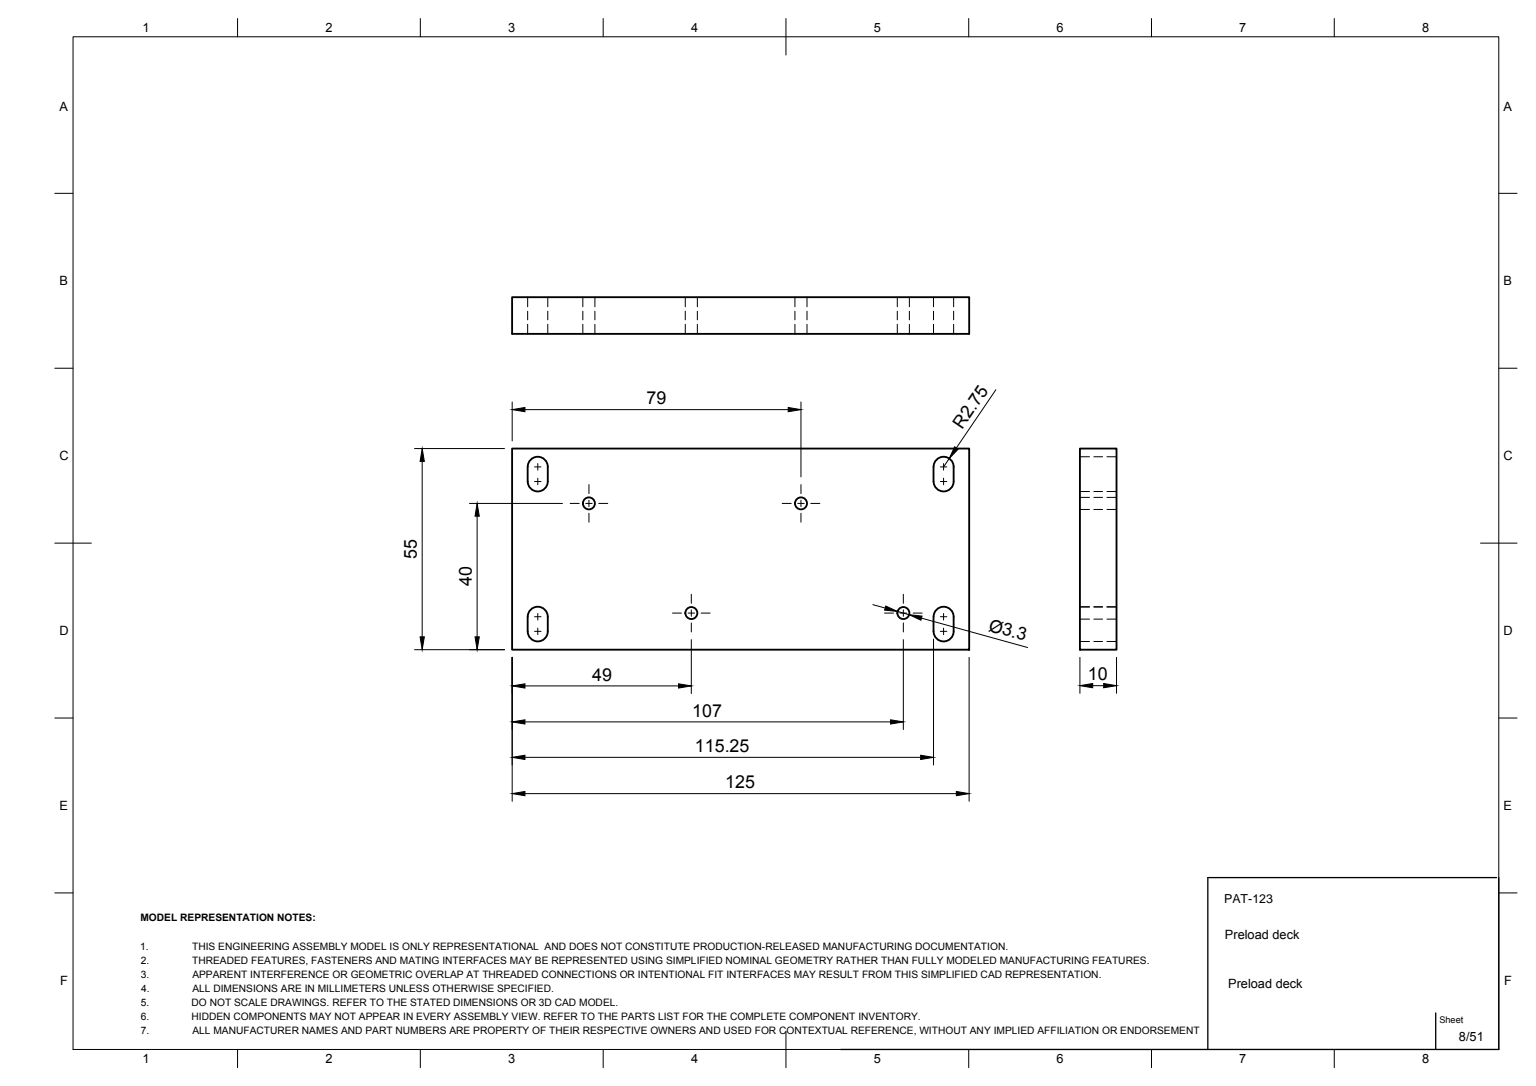
ISO-10303-21;
HEADER;
/* Generated by software containing ST-Developer
 * from STEP Tools, Inc. (www.steptools.com) 
 */

FILE_DESCRIPTION(
/* description */ ('Worm-less right-angle friction wheel drive'),
/* implementation_level */ '2;1');

FILE_NAME(
/* name */ 'Preload deck.step',
/* time_stamp */ '2026-10-28T03:22:36-07:00',
/* author */ (''),
/* organization */ (''),
/* preprocessor_version */ 'ST-DEVELOPER v20.2',
/* originating_system */ 'Autodesk Translation Framework v15.17.0.0',
/* authorisation */ '');

FILE_SCHEMA (('AUTOMOTIVE_DESIGN { 1 0 10303 214 3 1 1 }'));
ENDSEC;

DATA;
#10=MECHANICAL_DESIGN_GEOMETRIC_PRESENTATION_REPRESENTATION('',(#614),#17046);
#520=SHAPE_REPRESENTATION_RELATIONSHIP('SRR','None',#17263,#567);
#567=ADVANCED_BREP_SHAPE_REPRESENTATION('',(#668),#16999);
#614=STYLED_ITEM('',(#17584),#668);
#668=MANIFOLD_SOLID_BREP('Body1',#8169);
#735=FACE_BOUND('',#1729,.T.);
#736=FACE_BOUND('',#1730,.T.);
#737=FACE_BOUND('',#1731,.T.);
#738=FACE_BOUND('',#1732,.T.);
#739=FACE_BOUND('',#1733,.T.);
#740=FACE_BOUND('',#1734,.T.);
#741=FACE_BOUND('',#1735,.T.);
#742=FACE_BOUND('',#1736,.T.);
#743=FACE_BOUND('',#1756,.T.);
#744=FACE_BOUND('',#1757,.T.);
#745=FACE_BOUND('',#1758,.T.);
#746=FACE_BOUND('',#1759,.T.);
#747=FACE_BOUND('',#1760,.T.);
#748=FACE_BOUND('',#1761,.T.);
#749=FACE_BOUND('',#1762,.T.);
#750=FACE_BOUND('',#1763,.T.);
#970=PLANE('',#8814);
#971=PLANE('',#8821);
#972=PLANE('',#8822);
#973=PLANE('',#8827);
#974=PLANE('',#8828);
#975=PLANE('',#8833);
#976=PLANE('',#8834);
#977=PLANE('',#8839);
#978=PLANE('',#8840);
#979=PLANE('',#8841);
#980=PLANE('',#8842);
#981=PLANE('',#8843);
#982=PLANE('',#8844);
#983=PLANE('',#8845);
#1236=FACE_OUTER_BOUND('',#1722,.T.);
#1237=FACE_OUTER_BOUND('',#1723,.T.);
#1238=FACE_OUTER_BOUND('',#1724,.T.);
#1239=FACE_OUTER_BOUND('',#1725,.T.);
#1240=FACE_OUTER_BOUND('',#1726,.T.);
#1241=FACE_OUTER_BOUND('',#1727,.T.);
#1242=FACE_OUTER_BOUND('',#1728,.T.);
#1243=FACE_OUTER_BOUND('',#1737,.T.);
#1244=FACE_OUTER_BOUND('',#1738,.T.);
#1245=FACE_OUTER_BOUND('',#1739,.T.);
#1246=FACE_OUTER_BOUND('',#1740,.T.);
#1247=FACE_OUTER_BOUND('',#1741,.T.);
#1248=FACE_OUTER_BOUND('',#1742,.T.);
#1249=FACE_OUTER_BOUND('',#1743,.T.);
#1250=FACE_OUTER_BOUND('',#1744,.T.);
#1251=FACE_OUTER_BOUND('',#1745,.T.);
#1252=FACE_OUTER_BOUND('',#1746,.T.);
#1253=FACE_OUTER_BOUND('',#1747,.T.);
#1254=FACE_OUTER_BOUND('',#1748,.T.);
#1255=FACE_OUTER_BOUND('',#1749,.T.);
#1256=FACE_OUTER_BOUND('',#1750,.T.);
#1257=FACE_OUTER_BOUND('',#1751,.T.);
#1258=FACE_OUTER_BOUND('',#1752,.T.);
#1259=FACE_OUTER_BOUND('',#1753,.T.);
#1260=FACE_OUTER_BOUND('',#1754,.T.);
#1261=FACE_OUTER_BOUND('',#1755,.T.);
#1722=EDGE_LOOP('',(#5666,#5667,#5668,#5669));
#1723=EDGE_LOOP('',(#5670,#5671,#5672,#5673));
#1724=EDGE_LOOP('',(#5674,#5675,#5676,#5677));
#1725=EDGE_LOOP('',(#5678,#5679,#5680,#5681));
#1726=EDGE_LOOP('',(#5682,#5683,#5684,#5685));
#1727=EDGE_LOOP('',(#5686,#5687,#5688,#5689));
#1728=EDGE_LOOP('',(#5690,#5691,#5692,#5693));
#1729=EDGE_LOOP('',(#5694,#5695,#5696,#5697));
#1730=EDGE_LOOP('',(#5698,#5699,#5700,#5701));
#1731=EDGE_LOOP('',(#5702,#5703,#5704,#5705));
#1732=EDGE_LOOP('',(#5706,#5707,#5708,#5709));
#1733=EDGE_LOOP('',(#5710));
#1734=EDGE_LOOP('',(#5711));
#1735=EDGE_LOOP('',(#5712));
#1736=EDGE_LOOP('',(#5713));
#1737=EDGE_LOOP('',(#5714,#5715,#5716,#5717));
#1738=EDGE_LOOP('',(#5718,#5719,#5720,#5721));
#1739=EDGE_LOOP('',(#5722,#5723,#5724,#5725));
#1740=EDGE_LOOP('',(#5726,#5727,#5728,#5729));
#1741=EDGE_LOOP('',(#5730,#5731,#5732,#5733));
#1742=EDGE_LOOP('',(#5734,#5735,#5736,#5737));
#1743=EDGE_LOOP('',(#5738,#5739,#5740,#5741));
#1744=EDGE_LOOP('',(#5742,#5743,#5744,#5745));
#1745=EDGE_LOOP('',(#5746,#5747,#5748,#5749));
#1746=EDGE_LOOP('',(#5750,#5751,#5752,#5753));
#1747=EDGE_LOOP('',(#5754,#5755,#5756,#5757));
#1748=EDGE_LOOP('',(#5758,#5759,#5760,#5761));
#1749=EDGE_LOOP('',(#5762,#5763,#5764,#5765));
#1750=EDGE_LOOP('',(#5766,#5767,#5768,#5769));
#1751=EDGE_LOOP('',(#5770,#5771,#5772,#5773));
#1752=EDGE_LOOP('',(#5774,#5775,#5776,#5777));
#1753=EDGE_LOOP('',(#5778,#5779,#5780,#5781));
#1754=EDGE_LOOP('',(#5782,#5783,#5784,#5785));
#1755=EDGE_LOOP('',(#5786,#5787,#5788,#5789));
#1756=EDGE_LOOP('',(#5790,#5791,#5792,#5793));
#1757=EDGE_LOOP('',(#5794,#5795,#5796,#5797));
#1758=EDGE_LOOP('',(#5798,#5799,#5800,#5801));
#1759=EDGE_LOOP('',(#5802,#5803,#5804,#5805));
#1760=EDGE_LOOP('',(#5806));
#1761=EDGE_LOOP('',(#5807));
#1762=EDGE_LOOP('',(#5808));
#1763=EDGE_LOOP('',(#5809));
#2423=LINE('',#12523,#2963);
#2424=LINE('',#12529,#2964);
#2425=LINE('',#12535,#2965);
#2426=LINE('',#12541,#2966);
#2427=LINE('',#12546,#2967);
#2428=LINE('',#12550,#2968);
#2429=LINE('',#12555,#2969);
#2430=LINE('',#12559,#2970);
#2431=LINE('',#12564,#2971);
#2432=LINE('',#12566,#2972);
#2433=LINE('',#12568,#2973);
#2434=LINE('',#12569,#2974);
#2435=LINE('',#12570,#2975);
#2436=LINE('',#12571,#2976);
#2437=LINE('',#12576,#2977);
#2438=LINE('',#12579,#2978);
#2439=LINE('',#12584,#2979);
#2440=LINE('',#12587,#2980);
#2441=LINE('',#12592,#2981);
#2442=LINE('',#12595,#2982);
#2443=LINE('',#12597,#2983);
#2444=LINE('',#12599,#2984);
#2445=LINE('',#12602,#2985);
#2446=LINE('',#12604,#2986);
#2447=LINE('',#12608,#2987);
#2448=LINE('',#12610,#2988);
#2449=LINE('',#12613,#2989);
#2450=LINE('',#12615,#2990);
#2451=LINE('',#12618,#2991);
#2452=LINE('',#12620,#2992);
#2453=LINE('',#12624,#2993);
#2454=LINE('',#12626,#2994);
#2455=LINE('',#12629,#2995);
#2456=LINE('',#12631,#2996);
#2457=LINE('',#12634,#2997);
#2458=LINE('',#12636,#2998);
#2459=LINE('',#12640,#2999);
#2460=LINE('',#12642,#3000);
#2461=LINE('',#12645,#3001);
#2462=LINE('',#12647,#3002);
#2463=LINE('',#12651,#3003);
#2464=LINE('',#12652,#3004);
#2465=LINE('',#12653,#3005);
#2466=LINE('',#12656,#3006);
#2467=LINE('',#12657,#3007);
#2468=LINE('',#12660,#3008);
#2469=LINE('',#12661,#3009);
#2470=LINE('',#12663,#3010);
#2963=VECTOR('',#9931,0.165);
#2964=VECTOR('',#9938,0.165);
#2965=VECTOR('',#9945,0.165);
#2966=VECTOR('',#9952,0.165);
#2967=VECTOR('',#9957,1.);
#2968=VECTOR('',#9960,1.);
#2969=VECTOR('',#9965,1.);
#2970=VECTOR('',#9968,1.);
#2971=VECTOR('',#9973,1.);
#2972=VECTOR('',#9974,1.);
#2973=VECTOR('',#9975,1.);
#2974=VECTOR('',#9976,1.);
#2975=VECTOR('',#9977,1.);
#2976=VECTOR('',#9978,1.);
#2977=VECTOR('',#9981,1.);
#2978=VECTOR('',#9984,1.);
#2979=VECTOR('',#9987,1.);
#2980=VECTOR('',#9990,1.);
#2981=VECTOR('',#9993,1.);
#2982=VECTOR('',#9996,1.);
#2983=VECTOR('',#9999,1.);
#2984=VECTOR('',#10002,1.);
#2985=VECTOR('',#10005,1.);
#2986=VECTOR('',#10006,1.);
#2987=VECTOR('',#10011,1.);
#2988=VECTOR('',#10012,1.);
#2989=VECTOR('',#10017,1.);
#2990=VECTOR('',#10020,1.);
#2991=VECTOR('',#10023,1.);
#2992=VECTOR('',#10024,1.);
#2993=VECTOR('',#10029,1.);
#2994=VECTOR('',#10030,1.);
#2995=VECTOR('',#10035,1.);
#2996=VECTOR('',#10038,1.);
#2997=VECTOR('',#10041,1.);
#2998=VECTOR('',#10042,1.);
#2999=VECTOR('',#10047,1.);
#3000=VECTOR('',#10048,1.);
#3001=VECTOR('',#10053,1.);
#3002=VECTOR('',#10056,1.);
#3003=VECTOR('',#10059,1.);
#3004=VECTOR('',#10060,1.);
#3005=VECTOR('',#10061,1.);
#3006=VECTOR('',#10064,1.);
#3007=VECTOR('',#10065,1.);
#3008=VECTOR('',#10068,1.);
#3009=VECTOR('',#10069,1.);
#3010=VECTOR('',#10072,1.);
#3477=CIRCLE('',#8797,0.165);
#3478=CIRCLE('',#8798,0.165);
#3479=CIRCLE('',#8800,0.165);
#3480=CIRCLE('',#8801,0.165);
#3481=CIRCLE('',#8803,0.165);
#3482=CIRCLE('',#8804,0.165);
#3483=CIRCLE('',#8806,0.165);
#3484=CIRCLE('',#8807,0.165);
#3485=CIRCLE('',#8809,0.275);
#3486=CIRCLE('',#8810,0.275);
#3487=CIRCLE('',#8812,0.275);
#3488=CIRCLE('',#8813,0.275);
#3489=CIRCLE('',#8815,0.275);
#3490=CIRCLE('',#8816,0.275);
#3491=CIRCLE('',#8817,0.275);
#3492=CIRCLE('',#8818,0.275);
#3493=CIRCLE('',#8819,0.275);
#3494=CIRCLE('',#8820,0.275);
#3495=CIRCLE('',#8824,0.275);
#3496=CIRCLE('',#8826,0.275);
#3497=CIRCLE('',#8830,0.275);
#3498=CIRCLE('',#8832,0.275);
#3499=CIRCLE('',#8836,0.275);
#3500=CIRCLE('',#8838,0.275);
#3913=VERTEX_POINT('',#12520);
#3914=VERTEX_POINT('',#12522);
#3915=VERTEX_POINT('',#12526);
#3916=VERTEX_POINT('',#12528);
#3917=VERTEX_POINT('',#12532);
#3918=VERTEX_POINT('',#12534);
#3919=VERTEX_POINT('',#12538);
#3920=VERTEX_POINT('',#12540);
#3921=VERTEX_POINT('',#12544);
#3922=VERTEX_POINT('',#12545);
#3923=VERTEX_POINT('',#12547);
#3924=VERTEX_POINT('',#12549);
#3925=VERTEX_POINT('',#12553);
#3926=VERTEX_POINT('',#12554);
#3927=VERTEX_POINT('',#12556);
#3928=VERTEX_POINT('',#12558);
#3929=VERTEX_POINT('',#12562);
#3930=VERTEX_POINT('',#12563);
#3931=VERTEX_POINT('',#12565);
#3932=VERTEX_POINT('',#12567);
#3933=VERTEX_POINT('',#12572);
#3934=VERTEX_POINT('',#12573);
#3935=VERTEX_POINT('',#12575);
#3936=VERTEX_POINT('',#12577);
#3937=VERTEX_POINT('',#12580);
#3938=VERTEX_POINT('',#12581);
#3939=VERTEX_POINT('',#12583);
#3940=VERTEX_POINT('',#12585);
#3941=VERTEX_POINT('',#12588);
#3942=VERTEX_POINT('',#12589);
#3943=VERTEX_POINT('',#12591);
#3944=VERTEX_POINT('',#12593);
#3945=VERTEX_POINT('',#12601);
#3946=VERTEX_POINT('',#12603);
#3947=VERTEX_POINT('',#12607);
#3948=VERTEX_POINT('',#12609);
#3949=VERTEX_POINT('',#12617);
#3950=VERTEX_POINT('',#12619);
#3951=VERTEX_POINT('',#12623);
#3952=VERTEX_POINT('',#12625);
#3953=VERTEX_POINT('',#12633);
#3954=VERTEX_POINT('',#12635);
#3955=VERTEX_POINT('',#12639);
#3956=VERTEX_POINT('',#12641);
#3957=VERTEX_POINT('',#12649);
#3958=VERTEX_POINT('',#12650);
#3959=VERTEX_POINT('',#12655);
#3960=VERTEX_POINT('',#12659);
#4602=EDGE_CURVE('',#3913,#3913,#3477,.T.);
#4603=EDGE_CURVE('',#3913,#3914,#2423,.T.);
#4604=EDGE_CURVE('',#3914,#3914,#3478,.T.);
#4605=EDGE_CURVE('',#3915,#3915,#3479,.T.);
#4606=EDGE_CURVE('',#3915,#3916,#2424,.T.);
#4607=EDGE_CURVE('',#3916,#3916,#3480,.T.);
#4608=EDGE_CURVE('',#3917,#3917,#3481,.T.);
#4609=EDGE_CURVE('',#3917,#3918,#2425,.T.);
#4610=EDGE_CURVE('',#3918,#3918,#3482,.T.);
#4611=EDGE_CURVE('',#3919,#3919,#3483,.T.);
#4612=EDGE_CURVE('',#3919,#3920,#2426,.T.);
#4613=EDGE_CURVE('',#3920,#3920,#3484,.T.);
#4614=EDGE_CURVE('',#3921,#3922,#2427,.T.);
#4615=EDGE_CURVE('',#3923,#3922,#3485,.T.);
#4616=EDGE_CURVE('',#3924,#3923,#2428,.T.);
#4617=EDGE_CURVE('',#3921,#3924,#3486,.T.);
#4618=EDGE_CURVE('',#3925,#3926,#2429,.T.);
#4619=EDGE_CURVE('',#3927,#3926,#3487,.T.);
#4620=EDGE_CURVE('',#3928,#3927,#2430,.T.);
#4621=EDGE_CURVE('',#3925,#3928,#3488,.T.);
#4622=EDGE_CURVE('',#3929,#3930,#2431,.T.);
#4623=EDGE_CURVE('',#3930,#3931,#2432,.T.);
#4624=EDGE_CURVE('',#3931,#3932,#2433,.T.);
#4625=EDGE_CURVE('',#3932,#3929,#2434,.T.);
#4626=EDGE_CURVE('',#3922,#3927,#2435,.T.);
#4627=EDGE_CURVE('',#3926,#3923,#2436,.T.);
#4628=EDGE_CURVE('',#3933,#3934,#3489,.T.);
#4629=EDGE_CURVE('',#3934,#3935,#2437,.T.);
#4630=EDGE_CURVE('',#3935,#3936,#3490,.T.);
#4631=EDGE_CURVE('',#3936,#3933,#2438,.T.);
#4632=EDGE_CURVE('',#3937,#3938,#3491,.T.);
#4633=EDGE_CURVE('',#3938,#3939,#2439,.T.);
#4634=EDGE_CURVE('',#3939,#3940,#3492,.T.);
#4635=EDGE_CURVE('',#3940,#3937,#2440,.T.);
#4636=EDGE_CURVE('',#3941,#3942,#3493,.T.);
#4637=EDGE_CURVE('',#3942,#3943,#2441,.T.);
#4638=EDGE_CURVE('',#3943,#3944,#3494,.T.);
#4639=EDGE_CURVE('',#3944,#3941,#2442,.T.);
#4640=EDGE_CURVE('',#3928,#3921,#2443,.T.);
#4641=EDGE_CURVE('',#3924,#3925,#2444,.T.);
#4642=EDGE_CURVE('',#3945,#3942,#2445,.T.);
#4643=EDGE_CURVE('',#3946,#3941,#2446,.T.);
#4644=EDGE_CURVE('',#3945,#3946,#3495,.T.);
#4645=EDGE_CURVE('',#3947,#3944,#2447,.T.);
#4646=EDGE_CURVE('',#3948,#3943,#2448,.T.);
#4647=EDGE_CURVE('',#3947,#3948,#3496,.T.);
#4648=EDGE_CURVE('',#3948,#3945,#2449,.T.);
#4649=EDGE_CURVE('',#3946,#3947,#2450,.T.);
#4650=EDGE_CURVE('',#3949,#3934,#2451,.T.);
#4651=EDGE_CURVE('',#3950,#3933,#2452,.T.);
#4652=EDGE_CURVE('',#3949,#3950,#3497,.T.);
#4653=EDGE_CURVE('',#3951,#3936,#2453,.T.);
#4654=EDGE_CURVE('',#3952,#3935,#2454,.T.);
#4655=EDGE_CURVE('',#3951,#3952,#3498,.T.);
#4656=EDGE_CURVE('',#3952,#3949,#2455,.T.);
#4657=EDGE_CURVE('',#3950,#3951,#2456,.T.);
#4658=EDGE_CURVE('',#3953,#3938,#2457,.T.);
#4659=EDGE_CURVE('',#3954,#3937,#2458,.T.);
#4660=EDGE_CURVE('',#3953,#3954,#3499,.T.);
#4661=EDGE_CURVE('',#3955,#3940,#2459,.T.);
#4662=EDGE_CURVE('',#3956,#3939,#2460,.T.);
#4663=EDGE_CURVE('',#3955,#3956,#3500,.T.);
#4664=EDGE_CURVE('',#3956,#3953,#2461,.T.);
#4665=EDGE_CURVE('',#3954,#3955,#2462,.T.);
#4666=EDGE_CURVE('',#3957,#3958,#2463,.T.);
#4667=EDGE_CURVE('',#3958,#3929,#2464,.T.);
#4668=EDGE_CURVE('',#3957,#3932,#2465,.T.);
#4669=EDGE_CURVE('',#3959,#3957,#2466,.T.);
#4670=EDGE_CURVE('',#3959,#3931,#2467,.T.);
#4671=EDGE_CURVE('',#3960,#3959,#2468,.T.);
#4672=EDGE_CURVE('',#3960,#3930,#2469,.T.);
#4673=EDGE_CURVE('',#3958,#3960,#2470,.T.);
#5666=ORIENTED_EDGE('',*,*,#4602,.F.);
#5667=ORIENTED_EDGE('',*,*,#4603,.T.);
#5668=ORIENTED_EDGE('',*,*,#4604,.F.);
#5669=ORIENTED_EDGE('',*,*,#4603,.F.);
#5670=ORIENTED_EDGE('',*,*,#4605,.F.);
#5671=ORIENTED_EDGE('',*,*,#4606,.T.);
#5672=ORIENTED_EDGE('',*,*,#4607,.F.);
#5673=ORIENTED_EDGE('',*,*,#4606,.F.);
#5674=ORIENTED_EDGE('',*,*,#4608,.F.);
#5675=ORIENTED_EDGE('',*,*,#4609,.T.);
#5676=ORIENTED_EDGE('',*,*,#4610,.F.);
#5677=ORIENTED_EDGE('',*,*,#4609,.F.);
#5678=ORIENTED_EDGE('',*,*,#4611,.F.);
#5679=ORIENTED_EDGE('',*,*,#4612,.T.);
#5680=ORIENTED_EDGE('',*,*,#4613,.F.);
#5681=ORIENTED_EDGE('',*,*,#4612,.F.);
#5682=ORIENTED_EDGE('',*,*,#4614,.T.);
#5683=ORIENTED_EDGE('',*,*,#4615,.F.);
#5684=ORIENTED_EDGE('',*,*,#4616,.F.);
#5685=ORIENTED_EDGE('',*,*,#4617,.F.);
#5686=ORIENTED_EDGE('',*,*,#4618,.T.);
#5687=ORIENTED_EDGE('',*,*,#4619,.F.);
#5688=ORIENTED_EDGE('',*,*,#4620,.F.);
#5689=ORIENTED_EDGE('',*,*,#4621,.F.);
#5690=ORIENTED_EDGE('',*,*,#4622,.T.);
#5691=ORIENTED_EDGE('',*,*,#4623,.T.);
#5692=ORIENTED_EDGE('',*,*,#4624,.T.);
#5693=ORIENTED_EDGE('',*,*,#4625,.T.);
#5694=ORIENTED_EDGE('',*,*,#4615,.T.);
#5695=ORIENTED_EDGE('',*,*,#4626,.T.);
#5696=ORIENTED_EDGE('',*,*,#4619,.T.);
#5697=ORIENTED_EDGE('',*,*,#4627,.T.);
#5698=ORIENTED_EDGE('',*,*,#4628,.T.);
#5699=ORIENTED_EDGE('',*,*,#4629,.T.);
#5700=ORIENTED_EDGE('',*,*,#4630,.T.);
#5701=ORIENTED_EDGE('',*,*,#4631,.T.);
#5702=ORIENTED_EDGE('',*,*,#4632,.T.);
#5703=ORIENTED_EDGE('',*,*,#4633,.T.);
#5704=ORIENTED_EDGE('',*,*,#4634,.T.);
#5705=ORIENTED_EDGE('',*,*,#4635,.T.);
#5706=ORIENTED_EDGE('',*,*,#4636,.T.);
#5707=ORIENTED_EDGE('',*,*,#4637,.T.);
#5708=ORIENTED_EDGE('',*,*,#4638,.T.);
#5709=ORIENTED_EDGE('',*,*,#4639,.T.);
#5710=ORIENTED_EDGE('',*,*,#4613,.T.);
#5711=ORIENTED_EDGE('',*,*,#4610,.T.);
#5712=ORIENTED_EDGE('',*,*,#4607,.T.);
#5713=ORIENTED_EDGE('',*,*,#4604,.T.);
#5714=ORIENTED_EDGE('',*,*,#4626,.F.);
#5715=ORIENTED_EDGE('',*,*,#4614,.F.);
#5716=ORIENTED_EDGE('',*,*,#4640,.F.);
#5717=ORIENTED_EDGE('',*,*,#4620,.T.);
#5718=ORIENTED_EDGE('',*,*,#4627,.F.);
#5719=ORIENTED_EDGE('',*,*,#4618,.F.);
#5720=ORIENTED_EDGE('',*,*,#4641,.F.);
#5721=ORIENTED_EDGE('',*,*,#4616,.T.);
#5722=ORIENTED_EDGE('',*,*,#4642,.T.);
#5723=ORIENTED_EDGE('',*,*,#4636,.F.);
#5724=ORIENTED_EDGE('',*,*,#4643,.F.);
#5725=ORIENTED_EDGE('',*,*,#4644,.F.);
#5726=ORIENTED_EDGE('',*,*,#4645,.T.);
#5727=ORIENTED_EDGE('',*,*,#4638,.F.);
#5728=ORIENTED_EDGE('',*,*,#4646,.F.);
#5729=ORIENTED_EDGE('',*,*,#4647,.F.);
#5730=ORIENTED_EDGE('',*,*,#4637,.F.);
#5731=ORIENTED_EDGE('',*,*,#4642,.F.);
#5732=ORIENTED_EDGE('',*,*,#4648,.F.);
#5733=ORIENTED_EDGE('',*,*,#4646,.T.);
#5734=ORIENTED_EDGE('',*,*,#4639,.F.);
#5735=ORIENTED_EDGE('',*,*,#4645,.F.);
#5736=ORIENTED_EDGE('',*,*,#4649,.F.);
#5737=ORIENTED_EDGE('',*,*,#4643,.T.);
#5738=ORIENTED_EDGE('',*,*,#4650,.T.);
#5739=ORIENTED_EDGE('',*,*,#4628,.F.);
#5740=ORIENTED_EDGE('',*,*,#4651,.F.);
#5741=ORIENTED_EDGE('',*,*,#4652,.F.);
#5742=ORIENTED_EDGE('',*,*,#4653,.T.);
#5743=ORIENTED_EDGE('',*,*,#4630,.F.);
#5744=ORIENTED_EDGE('',*,*,#4654,.F.);
#5745=ORIENTED_EDGE('',*,*,#4655,.F.);
#5746=ORIENTED_EDGE('',*,*,#4629,.F.);
#5747=ORIENTED_EDGE('',*,*,#4650,.F.);
#5748=ORIENTED_EDGE('',*,*,#4656,.F.);
#5749=ORIENTED_EDGE('',*,*,#4654,.T.);
#5750=ORIENTED_EDGE('',*,*,#4631,.F.);
#5751=ORIENTED_EDGE('',*,*,#4653,.F.);
#5752=ORIENTED_EDGE('',*,*,#4657,.F.);
#5753=ORIENTED_EDGE('',*,*,#4651,.T.);
#5754=ORIENTED_EDGE('',*,*,#4658,.T.);
#5755=ORIENTED_EDGE('',*,*,#4632,.F.);
#5756=ORIENTED_EDGE('',*,*,#4659,.F.);
#5757=ORIENTED_EDGE('',*,*,#4660,.F.);
#5758=ORIENTED_EDGE('',*,*,#4661,.T.);
#5759=ORIENTED_EDGE('',*,*,#4634,.F.);
#5760=ORIENTED_EDGE('',*,*,#4662,.F.);
#5761=ORIENTED_EDGE('',*,*,#4663,.F.);
#5762=ORIENTED_EDGE('',*,*,#4633,.F.);
#5763=ORIENTED_EDGE('',*,*,#4658,.F.);
#5764=ORIENTED_EDGE('',*,*,#4664,.F.);
#5765=ORIENTED_EDGE('',*,*,#4662,.T.);
#5766=ORIENTED_EDGE('',*,*,#4635,.F.);
#5767=ORIENTED_EDGE('',*,*,#4661,.F.);
#5768=ORIENTED_EDGE('',*,*,#4665,.F.);
#5769=ORIENTED_EDGE('',*,*,#4659,.T.);
#5770=ORIENTED_EDGE('',*,*,#4666,.T.);
#5771=ORIENTED_EDGE('',*,*,#4667,.T.);
#5772=ORIENTED_EDGE('',*,*,#4625,.F.);
#5773=ORIENTED_EDGE('',*,*,#4668,.F.);
#5774=ORIENTED_EDGE('',*,*,#4669,.T.);
#5775=ORIENTED_EDGE('',*,*,#4668,.T.);
#5776=ORIENTED_EDGE('',*,*,#4624,.F.);
#5777=ORIENTED_EDGE('',*,*,#4670,.F.);
#5778=ORIENTED_EDGE('',*,*,#4671,.T.);
#5779=ORIENTED_EDGE('',*,*,#4670,.T.);
#5780=ORIENTED_EDGE('',*,*,#4623,.F.);
#5781=ORIENTED_EDGE('',*,*,#4672,.F.);
#5782=ORIENTED_EDGE('',*,*,#4673,.T.);
#5783=ORIENTED_EDGE('',*,*,#4672,.T.);
#5784=ORIENTED_EDGE('',*,*,#4622,.F.);
#5785=ORIENTED_EDGE('',*,*,#4667,.F.);
#5786=ORIENTED_EDGE('',*,*,#4673,.F.);
#5787=ORIENTED_EDGE('',*,*,#4666,.F.);
#5788=ORIENTED_EDGE('',*,*,#4669,.F.);
#5789=ORIENTED_EDGE('',*,*,#4671,.F.);
#5790=ORIENTED_EDGE('',*,*,#4660,.T.);
#5791=ORIENTED_EDGE('',*,*,#4665,.T.);
#5792=ORIENTED_EDGE('',*,*,#4663,.T.);
#5793=ORIENTED_EDGE('',*,*,#4664,.T.);
#5794=ORIENTED_EDGE('',*,*,#4652,.T.);
#5795=ORIENTED_EDGE('',*,*,#4657,.T.);
#5796=ORIENTED_EDGE('',*,*,#4655,.T.);
#5797=ORIENTED_EDGE('',*,*,#4656,.T.);
#5798=ORIENTED_EDGE('',*,*,#4644,.T.);
#5799=ORIENTED_EDGE('',*,*,#4649,.T.);
#5800=ORIENTED_EDGE('',*,*,#4647,.T.);
#5801=ORIENTED_EDGE('',*,*,#4648,.T.);
#5802=ORIENTED_EDGE('',*,*,#4617,.T.);
#5803=ORIENTED_EDGE('',*,*,#4641,.T.);
#5804=ORIENTED_EDGE('',*,*,#4621,.T.);
#5805=ORIENTED_EDGE('',*,*,#4640,.T.);
#5806=ORIENTED_EDGE('',*,*,#4611,.T.);
#5807=ORIENTED_EDGE('',*,*,#4608,.T.);
#5808=ORIENTED_EDGE('',*,*,#4605,.T.);
#5809=ORIENTED_EDGE('',*,*,#4602,.T.);
#7540=CYLINDRICAL_SURFACE('',#8796,0.165);
#7541=CYLINDRICAL_SURFACE('',#8799,0.165);
#7542=CYLINDRICAL_SURFACE('',#8802,0.165);
#7543=CYLINDRICAL_SURFACE('',#8805,0.165);
#7544=CYLINDRICAL_SURFACE('',#8808,0.275);
#7545=CYLINDRICAL_SURFACE('',#8811,0.275);
#7546=CYLINDRICAL_SURFACE('',#8823,0.275);
#7547=CYLINDRICAL_SURFACE('',#8825,0.275);
#7548=CYLINDRICAL_SURFACE('',#8829,0.275);
#7549=CYLINDRICAL_SURFACE('',#8831,0.275);
#7550=CYLINDRICAL_SURFACE('',#8835,0.275);
#7551=CYLINDRICAL_SURFACE('',#8837,0.275);
#7728=ADVANCED_FACE('',(#1236),#7540,.F.);
#7729=ADVANCED_FACE('',(#1237),#7541,.F.);
#7730=ADVANCED_FACE('',(#1238),#7542,.F.);
#7731=ADVANCED_FACE('',(#1239),#7543,.F.);
#7732=ADVANCED_FACE('',(#1240),#7544,.F.);
#7733=ADVANCED_FACE('',(#1241),#7545,.F.);
#7734=ADVANCED_FACE('',(#1242,#735,#736,#737,#738,#739,#740,#741,#742),
#970,.T.);
#7735=ADVANCED_FACE('',(#1243),#971,.F.);
#7736=ADVANCED_FACE('',(#1244),#972,.F.);
#7737=ADVANCED_FACE('',(#1245),#7546,.F.);
#7738=ADVANCED_FACE('',(#1246),#7547,.F.);
#7739=ADVANCED_FACE('',(#1247),#973,.F.);
#7740=ADVANCED_FACE('',(#1248),#974,.F.);
#7741=ADVANCED_FACE('',(#1249),#7548,.F.);
#7742=ADVANCED_FACE('',(#1250),#7549,.F.);
#7743=ADVANCED_FACE('',(#1251),#975,.F.);
#7744=ADVANCED_FACE('',(#1252),#976,.F.);
#7745=ADVANCED_FACE('',(#1253),#7550,.F.);
#7746=ADVANCED_FACE('',(#1254),#7551,.F.);
#7747=ADVANCED_FACE('',(#1255),#977,.F.);
#7748=ADVANCED_FACE('',(#1256),#978,.F.);
#7749=ADVANCED_FACE('',(#1257),#979,.T.);
#7750=ADVANCED_FACE('',(#1258),#980,.T.);
#7751=ADVANCED_FACE('',(#1259),#981,.T.);
#7752=ADVANCED_FACE('',(#1260),#982,.T.);
#7753=ADVANCED_FACE('',(#1261,#743,#744,#745,#746,#747,#748,#749,#750),
#983,.F.);
#8169=CLOSED_SHELL('',(#7728,#7729,#7730,#7731,#7732,#7733,#7734,#7735,
#7736,#7737,#7738,#7739,#7740,#7741,#7742,#7743,#7744,#7745,#7746,#7747,
#7748,#7749,#7750,#7751,#7752,#7753));
#8795=AXIS2_PLACEMENT_3D('',#12518,#9925,#9926);
#8796=AXIS2_PLACEMENT_3D('',#12519,#9927,#9928);
#8797=AXIS2_PLACEMENT_3D('',#12521,#9929,#9930);
#8798=AXIS2_PLACEMENT_3D('',#12524,#9932,#9933);
#8799=AXIS2_PLACEMENT_3D('',#12525,#9934,#9935);
#8800=AXIS2_PLACEMENT_3D('',#12527,#9936,#9937);
#8801=AXIS2_PLACEMENT_3D('',#12530,#9939,#9940);
#8802=AXIS2_PLACEMENT_3D('',#12531,#9941,#9942);
#8803=AXIS2_PLACEMENT_3D('',#12533,#9943,#9944);
#8804=AXIS2_PLACEMENT_3D('',#12536,#9946,#9947);
#8805=AXIS2_PLACEMENT_3D('',#12537,#9948,#9949);
#8806=AXIS2_PLACEMENT_3D('',#12539,#9950,#9951);
#8807=AXIS2_PLACEMENT_3D('',#12542,#9953,#9954);
#8808=AXIS2_PLACEMENT_3D('',#12543,#9955,#9956);
#8809=AXIS2_PLACEMENT_3D('',#12548,#9958,#9959);
#8810=AXIS2_PLACEMENT_3D('',#12551,#9961,#9962);
#8811=AXIS2_PLACEMENT_3D('',#12552,#9963,#9964);
#8812=AXIS2_PLACEMENT_3D('',#12557,#9966,#9967);
#8813=AXIS2_PLACEMENT_3D('',#12560,#9969,#9970);
#8814=AXIS2_PLACEMENT_3D('',#12561,#9971,#9972);
#8815=AXIS2_PLACEMENT_3D('',#12574,#9979,#9980);
#8816=AXIS2_PLACEMENT_3D('',#12578,#9982,#9983);
#8817=AXIS2_PLACEMENT_3D('',#12582,#9985,#9986);
#8818=AXIS2_PLACEMENT_3D('',#12586,#9988,#9989);
#8819=AXIS2_PLACEMENT_3D('',#12590,#9991,#9992);
#8820=AXIS2_PLACEMENT_3D('',#12594,#9994,#9995);
#8821=AXIS2_PLACEMENT_3D('',#12596,#9997,#9998);
#8822=AXIS2_PLACEMENT_3D('',#12598,#10000,#10001);
#8823=AXIS2_PLACEMENT_3D('',#12600,#10003,#10004);
#8824=AXIS2_PLACEMENT_3D('',#12605,#10007,#10008);
#8825=AXIS2_PLACEMENT_3D('',#12606,#10009,#10010);
#8826=AXIS2_PLACEMENT_3D('',#12611,#10013,#10014);
#8827=AXIS2_PLACEMENT_3D('',#12612,#10015,#10016);
#8828=AXIS2_PLACEMENT_3D('',#12614,#10018,#10019);
#8829=AXIS2_PLACEMENT_3D('',#12616,#10021,#10022);
#8830=AXIS2_PLACEMENT_3D('',#12621,#10025,#10026);
#8831=AXIS2_PLACEMENT_3D('',#12622,#10027,#10028);
#8832=AXIS2_PLACEMENT_3D('',#12627,#10031,#10032);
#8833=AXIS2_PLACEMENT_3D('',#12628,#10033,#10034);
#8834=AXIS2_PLACEMENT_3D('',#12630,#10036,#10037);
#8835=AXIS2_PLACEMENT_3D('',#12632,#10039,#10040);
#8836=AXIS2_PLACEMENT_3D('',#12637,#10043,#10044);
#8837=AXIS2_PLACEMENT_3D('',#12638,#10045,#10046);
#8838=AXIS2_PLACEMENT_3D('',#12643,#10049,#10050);
#8839=AXIS2_PLACEMENT_3D('',#12644,#10051,#10052);
#8840=AXIS2_PLACEMENT_3D('',#12646,#10054,#10055);
#8841=AXIS2_PLACEMENT_3D('',#12648,#10057,#10058);
#8842=AXIS2_PLACEMENT_3D('',#12654,#10062,#10063);
#8843=AXIS2_PLACEMENT_3D('',#12658,#10066,#10067);
#8844=AXIS2_PLACEMENT_3D('',#12662,#10070,#10071);
#8845=AXIS2_PLACEMENT_3D('',#12664,#10073,#10074);
#9925=DIRECTION('axis',(0.,0.,1.));
#9926=DIRECTION('refdir',(1.,0.,0.));
#9927=DIRECTION('center_axis',(0.,0.,1.));
#9928=DIRECTION('ref_axis',(1.,0.,0.));
#9929=DIRECTION('center_axis',(0.,0.,1.));
#9930=DIRECTION('ref_axis',(1.,0.,0.));
#9931=DIRECTION('',(0.,0.,1.));
#9932=DIRECTION('center_axis',(0.,0.,-1.));
#9933=DIRECTION('ref_axis',(1.,0.,0.));
#9934=DIRECTION('center_axis',(0.,0.,1.));
#9935=DIRECTION('ref_axis',(1.,0.,0.));
#9936=DIRECTION('center_axis',(0.,0.,1.));
#9937=DIRECTION('ref_axis',(1.,0.,0.));
#9938=DIRECTION('',(0.,0.,1.));
#9939=DIRECTION('center_axis',(0.,0.,-1.));
#9940=DIRECTION('ref_axis',(1.,0.,0.));
#9941=DIRECTION('center_axis',(0.,0.,1.));
#9942=DIRECTION('ref_axis',(1.,0.,0.));
#9943=DIRECTION('center_axis',(0.,0.,1.));
#9944=DIRECTION('ref_axis',(1.,0.,0.));
#9945=DIRECTION('',(0.,0.,1.));
#9946=DIRECTION('center_axis',(0.,0.,-1.));
#9947=DIRECTION('ref_axis',(1.,0.,0.));
#9948=DIRECTION('center_axis',(0.,0.,1.));
#9949=DIRECTION('ref_axis',(1.,0.,0.));
#9950=DIRECTION('center_axis',(0.,0.,1.));
#9951=DIRECTION('ref_axis',(1.,0.,0.));
#9952=DIRECTION('',(0.,0.,1.));
#9953=DIRECTION('center_axis',(0.,0.,-1.));
#9954=DIRECTION('ref_axis',(1.,0.,0.));
#9955=DIRECTION('center_axis',(0.,0.,1.));
#9956=DIRECTION('ref_axis',(1.,0.,0.));
#9957=DIRECTION('',(0.,0.,1.));
#9958=DIRECTION('center_axis',(0.,0.,-1.));
#9959=DIRECTION('ref_axis',(1.,0.,0.));
#9960=DIRECTION('',(0.,0.,1.));
#9961=DIRECTION('center_axis',(0.,0.,1.));
#9962=DIRECTION('ref_axis',(1.,0.,0.));
#9963=DIRECTION('center_axis',(0.,0.,1.));
#9964=DIRECTION('ref_axis',(1.,0.,0.));
#9965=DIRECTION('',(0.,0.,1.));
#9966=DIRECTION('center_axis',(0.,0.,-1.));
#9967=DIRECTION('ref_axis',(1.,0.,0.));
#9968=DIRECTION('',(0.,0.,1.));
#9969=DIRECTION('center_axis',(0.,0.,1.));
#9970=DIRECTION('ref_axis',(1.,0.,0.));
#9971=DIRECTION('center_axis',(0.,0.,1.));
#9972=DIRECTION('ref_axis',(1.,0.,0.));
#9973=DIRECTION('',(0.,-1.,0.));
#9974=DIRECTION('',(1.,0.,0.));
#9975=DIRECTION('',(0.,1.,0.));
#9976=DIRECTION('',(-1.,0.,0.));
#9977=DIRECTION('',(0.,1.,0.));
#9978=DIRECTION('',(0.,-1.,0.));
#9979=DIRECTION('center_axis',(0.,0.,-1.));
#9980=DIRECTION('ref_axis',(1.,0.,0.));
#9981=DIRECTION('',(0.,1.,0.));
#9982=DIRECTION('center_axis',(0.,0.,-1.));
#9983=DIRECTION('ref_axis',(1.,0.,0.));
#9984=DIRECTION('',(0.,-1.,0.));
#9985=DIRECTION('center_axis',(0.,0.,-1.));
#9986=DIRECTION('ref_axis',(1.,0.,0.));
#9987=DIRECTION('',(0.,1.,0.));
#9988=DIRECTION('center_axis',(0.,0.,-1.));
#9989=DIRECTION('ref_axis',(1.,0.,0.));
#9990=DIRECTION('',(0.,-1.,0.));
#9991=DIRECTION('center_axis',(0.,0.,-1.));
#9992=DIRECTION('ref_axis',(1.,0.,0.));
#9993=DIRECTION('',(0.,1.,0.));
#9994=DIRECTION('center_axis',(0.,0.,-1.));
#9995=DIRECTION('ref_axis',(1.,0.,0.));
#9996=DIRECTION('',(0.,-1.,0.));
#9997=DIRECTION('center_axis',(-1.,0.,0.));
#9998=DIRECTION('ref_axis',(0.,-1.,0.));
#9999=DIRECTION('',(0.,-1.,0.));
#10000=DIRECTION('center_axis',(1.,0.,0.));
#10001=DIRECTION('ref_axis',(0.,1.,0.));
#10002=DIRECTION('',(0.,1.,0.));
#10003=DIRECTION('center_axis',(0.,0.,1.));
#10004=DIRECTION('ref_axis',(1.,0.,0.));
#10005=DIRECTION('',(0.,0.,1.));
#10006=DIRECTION('',(0.,0.,1.));
#10007=DIRECTION('center_axis',(0.,0.,1.));
#10008=DIRECTION('ref_axis',(1.,0.,0.));
#10009=DIRECTION('center_axis',(0.,0.,1.));
#10010=DIRECTION('ref_axis',(1.,0.,0.));
#10011=DIRECTION('',(0.,0.,1.));
#10012=DIRECTION('',(0.,0.,1.));
#10013=DIRECTION('center_axis',(0.,0.,1.));
#10014=DIRECTION('ref_axis',(1.,0.,0.));
#10015=DIRECTION('center_axis',(-1.,0.,0.));
#10016=DIRECTION('ref_axis',(0.,-1.,0.));
#10017=DIRECTION('',(0.,-1.,0.));
#10018=DIRECTION('center_axis',(1.,0.,0.));
#10019=DIRECTION('ref_axis',(0.,1.,0.));
#10020=DIRECTION('',(0.,1.,0.));
#10021=DIRECTION('center_axis',(0.,0.,1.));
#10022=DIRECTION('ref_axis',(1.,0.,0.));
#10023=DIRECTION('',(0.,0.,1.));
#10024=DIRECTION('',(0.,0.,1.));
#10025=DIRECTION('center_axis',(0.,0.,1.));
#10026=DIRECTION('ref_axis',(1.,0.,0.));
#10027=DIRECTION('center_axis',(0.,0.,1.));
#10028=DIRECTION('ref_axis',(1.,0.,0.));
#10029=DIRECTION('',(0.,0.,1.));
#10030=DIRECTION('',(0.,0.,1.));
#10031=DIRECTION('center_axis',(0.,0.,1.));
#10032=DIRECTION('ref_axis',(1.,0.,0.));
#10033=DIRECTION('center_axis',(-1.,0.,0.));
#10034=DIRECTION('ref_axis',(0.,-1.,0.));
#10035=DIRECTION('',(0.,-1.,0.));
#10036=DIRECTION('center_axis',(1.,0.,0.));
#10037=DIRECTION('ref_axis',(0.,1.,0.));
#10038=DIRECTION('',(0.,1.,0.));
#10039=DIRECTION('center_axis',(0.,0.,1.));
#10040=DIRECTION('ref_axis',(1.,0.,0.));
#10041=DIRECTION('',(0.,0.,1.));
#10042=DIRECTION('',(0.,0.,1.));
#10043=DIRECTION('center_axis',(0.,0.,1.));
#10044=DIRECTION('ref_axis',(1.,0.,0.));
#10045=DIRECTION('center_axis',(0.,0.,1.));
#10046=DIRECTION('ref_axis',(1.,0.,0.));
#10047=DIRECTION('',(0.,0.,1.));
#10048=DIRECTION('',(0.,0.,1.));
#10049=DIRECTION('center_axis',(0.,0.,1.));
#10050=DIRECTION('ref_axis',(1.,0.,0.));
#10051=DIRECTION('center_axis',(-1.,0.,0.));
#10052=DIRECTION('ref_axis',(0.,-1.,0.));
#10053=DIRECTION('',(0.,-1.,0.));
#10054=DIRECTION('center_axis',(1.,0.,0.));
#10055=DIRECTION('ref_axis',(0.,1.,0.));
#10056=DIRECTION('',(0.,1.,0.));
#10057=DIRECTION('center_axis',(0.,1.,0.));
#10058=DIRECTION('ref_axis',(-1.,0.,0.));
#10059=DIRECTION('',(-1.,0.,0.));
#10060=DIRECTION('',(0.,0.,1.));
#10061=DIRECTION('',(0.,0.,1.));
#10062=DIRECTION('center_axis',(1.,0.,0.));
#10063=DIRECTION('ref_axis',(0.,1.,0.));
#10064=DIRECTION('',(0.,1.,0.));
#10065=DIRECTION('',(0.,0.,1.));
#10066=DIRECTION('center_axis',(0.,-1.,0.));
#10067=DIRECTION('ref_axis',(1.,0.,0.));
#10068=DIRECTION('',(1.,0.,0.));
#10069=DIRECTION('',(0.,0.,1.));
#10070=DIRECTION('center_axis',(-1.,0.,0.));
#10071=DIRECTION('ref_axis',(0.,-1.,0.));
#10072=DIRECTION('',(0.,-1.,0.));
#10073=DIRECTION('center_axis',(0.,0.,1.));
#10074=DIRECTION('ref_axis',(1.,0.,0.));
#12518=CARTESIAN_POINT('',(0.,0.,0.));
#12519=CARTESIAN_POINT('Origin',(4.1,1.5,0.9));
#12520=CARTESIAN_POINT('',(3.935,1.5,1.));
#12521=CARTESIAN_POINT('Origin',(4.1,1.5,1.));
#12522=CARTESIAN_POINT('',(3.935,1.5,2.));
#12523=CARTESIAN_POINT('',(3.935,1.5,0.9));
#12524=CARTESIAN_POINT('Origin',(4.1,1.5,2.));
#12525=CARTESIAN_POINT('Origin',(6.9,4.5,0.9));
#12526=CARTESIAN_POINT('',(6.735,4.5,1.));
#12527=CARTESIAN_POINT('Origin',(6.9,4.5,1.));
#12528=CARTESIAN_POINT('',(6.735,4.5,2.));
#12529=CARTESIAN_POINT('',(6.735,4.5,0.9));
#12530=CARTESIAN_POINT('Origin',(6.9,4.5,2.));
#12531=CARTESIAN_POINT('Origin',(-1.7,1.5,0.9));
#12532=CARTESIAN_POINT('',(-1.865,1.5,1.));
#12533=CARTESIAN_POINT('Origin',(-1.7,1.5,1.));
#12534=CARTESIAN_POINT('',(-1.865,1.5,2.));
#12535=CARTESIAN_POINT('',(-1.865,1.5,0.9));
#12536=CARTESIAN_POINT('Origin',(-1.7,1.5,2.));
#12537=CARTESIAN_POINT('Origin',(1.1,4.5,0.9));
#12538=CARTESIAN_POINT('',(0.935,4.5,1.));
#12539=CARTESIAN_POINT('Origin',(1.1,4.5,1.));
#12540=CARTESIAN_POINT('',(0.935,4.5,2.));
#12541=CARTESIAN_POINT('',(0.935,4.5,0.9));
#12542=CARTESIAN_POINT('Origin',(1.1,4.5,2.));
#12543=CARTESIAN_POINT('Origin',(8.3,5.1,0.9));
#12544=CARTESIAN_POINT('',(8.025,5.1,1.));
#12545=CARTESIAN_POINT('',(8.025,5.1,2.));
#12546=CARTESIAN_POINT('',(8.025,5.1,0.9));
#12547=CARTESIAN_POINT('',(8.575,5.1,2.));
#12548=CARTESIAN_POINT('Origin',(8.3,5.1,2.));
#12549=CARTESIAN_POINT('',(8.575,5.1,1.));
#12550=CARTESIAN_POINT('',(8.575,5.1,0.9));
#12551=CARTESIAN_POINT('Origin',(8.3,5.1,1.));
#12552=CARTESIAN_POINT('Origin',(8.3,5.5,0.9));
#12553=CARTESIAN_POINT('',(8.575,5.5,1.));
#12554=CARTESIAN_POINT('',(8.575,5.5,2.));
#12555=CARTESIAN_POINT('',(8.575,5.5,0.9));
#12556=CARTESIAN_POINT('',(8.025,5.5,2.));
#12557=CARTESIAN_POINT('Origin',(8.3,5.5,2.));
#12558=CARTESIAN_POINT('',(8.025,5.5,1.));
#12559=CARTESIAN_POINT('',(8.025,5.5,0.9));
#12560=CARTESIAN_POINT('Origin',(8.3,5.5,1.));
#12561=CARTESIAN_POINT('Origin',(2.75,3.25,2.));
#12562=CARTESIAN_POINT('',(-3.5,6.,2.));
#12563=CARTESIAN_POINT('',(-3.5,0.5,2.));
#12564=CARTESIAN_POINT('',(-3.5,6.,2.));
#12565=CARTESIAN_POINT('',(9.,0.5,2.));
#12566=CARTESIAN_POINT('',(-3.5,0.5,2.));
#12567=CARTESIAN_POINT('',(9.,6.,2.));
#12568=CARTESIAN_POINT('',(9.,0.5,2.));
#12569=CARTESIAN_POINT('',(9.,6.,2.));
#12570=CARTESIAN_POINT('',(8.025,4.375,2.));
#12571=CARTESIAN_POINT('',(8.575,4.175,2.));
#12572=CARTESIAN_POINT('',(-2.525,5.1,2.));
#12573=CARTESIAN_POINT('',(-3.075,5.1,2.));
#12574=CARTESIAN_POINT('Origin',(-2.8,5.1,2.));
#12575=CARTESIAN_POINT('',(-3.075,5.5,2.));
#12576=CARTESIAN_POINT('',(-3.075,4.375,2.));
#12577=CARTESIAN_POINT('',(-2.525,5.5,2.));
#12578=CARTESIAN_POINT('Origin',(-2.8,5.5,2.));
#12579=CARTESIAN_POINT('',(-2.525,4.175,2.));
#12580=CARTESIAN_POINT('',(-2.525,1.,2.));
#12581=CARTESIAN_POINT('',(-3.075,1.,2.));
#12582=CARTESIAN_POINT('Origin',(-2.8,1.,2.));
#12583=CARTESIAN_POINT('',(-3.075,1.4,2.));
#12584=CARTESIAN_POINT('',(-3.075,2.325,2.));
#12585=CARTESIAN_POINT('',(-2.525,1.4,2.));
#12586=CARTESIAN_POINT('Origin',(-2.8,1.4,2.));
#12587=CARTESIAN_POINT('',(-2.525,2.125,2.));
#12588=CARTESIAN_POINT('',(8.575,1.,2.));
#12589=CARTESIAN_POINT('',(8.025,1.,2.));
#12590=CARTESIAN_POINT('Origin',(8.3,1.,2.));
#12591=CARTESIAN_POINT('',(8.025,1.4,2.));
#12592=CARTESIAN_POINT('',(8.025,2.325,2.));
#12593=CARTESIAN_POINT('',(8.575,1.4,2.));
#12594=CARTESIAN_POINT('Origin',(8.3,1.4,2.));
#12595=CARTESIAN_POINT('',(8.575,2.125,2.));
#12596=CARTESIAN_POINT('Origin',(8.025,5.5,0.9));
#12597=CARTESIAN_POINT('',(8.025,4.375,1.));
#12598=CARTESIAN_POINT('Origin',(8.575,5.1,0.9));
#12599=CARTESIAN_POINT('',(8.575,4.175,1.));
#12600=CARTESIAN_POINT('Origin',(8.3,1.,0.9));
#12601=CARTESIAN_POINT('',(8.025,1.,1.));
#12602=CARTESIAN_POINT('',(8.025,1.,0.9));
#12603=CARTESIAN_POINT('',(8.575,1.,1.));
#12604=CARTESIAN_POINT('',(8.575,1.,0.9));
#12605=CARTESIAN_POINT('Origin',(8.3,1.,1.));
#12606=CARTESIAN_POINT('Origin',(8.3,1.4,0.9));
#12607=CARTESIAN_POINT('',(8.575,1.4,1.));
#12608=CARTESIAN_POINT('',(8.575,1.4,0.9));
#12609=CARTESIAN_POINT('',(8.025,1.4,1.));
#12610=CARTESIAN_POINT('',(8.025,1.4,0.9));
#12611=CARTESIAN_POINT('Origin',(8.3,1.4,1.));
#12612=CARTESIAN_POINT('Origin',(8.025,1.4,0.9));
#12613=CARTESIAN_POINT('',(8.025,2.325,1.));
#12614=CARTESIAN_POINT('Origin',(8.575,1.,0.9));
#12615=CARTESIAN_POINT('',(8.575,2.125,1.));
#12616=CARTESIAN_POINT('Origin',(-2.8,5.1,0.9));
#12617=CARTESIAN_POINT('',(-3.075,5.1,1.));
#12618=CARTESIAN_POINT('',(-3.075,5.1,0.9));
#12619=CARTESIAN_POINT('',(-2.525,5.1,1.));
#12620=CARTESIAN_POINT('',(-2.525,5.1,0.9));
#12621=CARTESIAN_POINT('Origin',(-2.8,5.1,1.));
#12622=CARTESIAN_POINT('Origin',(-2.8,5.5,0.9));
#12623=CARTESIAN_POINT('',(-2.525,5.5,1.));
#12624=CARTESIAN_POINT('',(-2.525,5.5,0.9));
#12625=CARTESIAN_POINT('',(-3.075,5.5,1.));
#12626=CARTESIAN_POINT('',(-3.075,5.5,0.9));
#12627=CARTESIAN_POINT('Origin',(-2.8,5.5,1.));
#12628=CARTESIAN_POINT('Origin',(-3.075,5.5,0.9));
#12629=CARTESIAN_POINT('',(-3.075,4.375,1.));
#12630=CARTESIAN_POINT('Origin',(-2.525,5.1,0.9));
#12631=CARTESIAN_POINT('',(-2.525,4.175,1.));
#12632=CARTESIAN_POINT('Origin',(-2.8,1.,0.9));
#12633=CARTESIAN_POINT('',(-3.075,1.,1.));
#12634=CARTESIAN_POINT('',(-3.075,1.,0.9));
#12635=CARTESIAN_POINT('',(-2.525,1.,1.));
#12636=CARTESIAN_POINT('',(-2.525,1.,0.9));
#12637=CARTESIAN_POINT('Origin',(-2.8,1.,1.));
#12638=CARTESIAN_POINT('Origin',(-2.8,1.4,0.9));
#12639=CARTESIAN_POINT('',(-2.525,1.4,1.));
#12640=CARTESIAN_POINT('',(-2.525,1.4,0.9));
#12641=CARTESIAN_POINT('',(-3.075,1.4,1.));
#12642=CARTESIAN_POINT('',(-3.075,1.4,0.9));
#12643=CARTESIAN_POINT('Origin',(-2.8,1.4,1.));
#12644=CARTESIAN_POINT('Origin',(-3.075,1.4,0.9));
#12645=CARTESIAN_POINT('',(-3.075,2.325,1.));
#12646=CARTESIAN_POINT('Origin',(-2.525,1.,0.9));
#12647=CARTESIAN_POINT('',(-2.525,2.125,1.));
#12648=CARTESIAN_POINT('Origin',(9.,6.,1.));
#12649=CARTESIAN_POINT('',(9.,6.,1.));
#12650=CARTESIAN_POINT('',(-3.5,6.,1.));
#12651=CARTESIAN_POINT('',(9.,6.,1.));
#12652=CARTESIAN_POINT('',(-3.5,6.,1.));
#12653=CARTESIAN_POINT('',(9.,6.,1.));
#12654=CARTESIAN_POINT('Origin',(9.,0.5,1.));
#12655=CARTESIAN_POINT('',(9.,0.5,1.));
#12656=CARTESIAN_POINT('',(9.,0.5,1.));
#12657=CARTESIAN_POINT('',(9.,0.5,1.));
#12658=CARTESIAN_POINT('Origin',(-3.5,0.5,1.));
#12659=CARTESIAN_POINT('',(-3.5,0.5,1.));
#12660=CARTESIAN_POINT('',(-3.5,0.5,1.));
#12661=CARTESIAN_POINT('',(-3.5,0.5,1.));
#12662=CARTESIAN_POINT('Origin',(-3.5,6.,1.));
#12663=CARTESIAN_POINT('',(-3.5,6.,1.));
#12664=CARTESIAN_POINT('Origin',(2.75,3.25,1.));
#16946=UNCERTAINTY_MEASURE_WITH_UNIT(LENGTH_MEASURE(0.001),#17047,
'DISTANCE_ACCURACY_VALUE',
'Maximum model space distance between geometric entities at asserted c
onnectivities');
#16993=UNCERTAINTY_MEASURE_WITH_UNIT(LENGTH_MEASURE(0.001),#17047,
'DISTANCE_ACCURACY_VALUE',
'Maximum model space distance between geometric entities at asserted c
onnectivities');
#16999=(
GEOMETRIC_REPRESENTATION_CONTEXT(3)
GLOBAL_UNCERTAINTY_ASSIGNED_CONTEXT((#16946))
GLOBAL_UNIT_ASSIGNED_CONTEXT((#17047,#17049,#17050))
REPRESENTATION_CONTEXT('','3D')
);
#17046=(
GEOMETRIC_REPRESENTATION_CONTEXT(3)
GLOBAL_UNCERTAINTY_ASSIGNED_CONTEXT((#16993))
GLOBAL_UNIT_ASSIGNED_CONTEXT((#17047,#17049,#17050))
REPRESENTATION_CONTEXT('','3D')
);
#17047=(
LENGTH_UNIT()
NAMED_UNIT(*)
SI_UNIT(.CENTI.,.METRE.)
);
#17049=(
NAMED_UNIT(*)
PLANE_ANGLE_UNIT()
SI_UNIT($,.RADIAN.)
);
#17050=(
NAMED_UNIT(*)
SI_UNIT($,.STERADIAN.)
SOLID_ANGLE_UNIT()
);
#17056=SHAPE_DEFINITION_REPRESENTATION(#17108,#17263);
#17108=PRODUCT_DEFINITION_SHAPE('',$,#17316);
#17263=SHAPE_REPRESENTATION('',(#8795),#16999);
#17310=PRODUCT_DEFINITION_CONTEXT('part definition',#17468,'design');
#17316=PRODUCT_DEFINITION('Preload deck','Preload deck',#17368,#17310);
#17368=PRODUCT_DEFINITION_FORMATION('',$,#17475);
#17468=APPLICATION_CONTEXT(
'Core Data for Automotive Mechanical Design Process');
#17469=PRODUCT_CONTEXT('part definition',#17468,'mechanical');
#17475=PRODUCT('Preload deck','Preload deck','Preload deck',(#17469));
#17578=COLOUR_RGB('Sky Blue',0.24,0.69,0.87);
#17579=FILL_AREA_STYLE_COLOUR('',#17578);
#17580=FILL_AREA_STYLE('',(#17579));
#17581=SURFACE_STYLE_FILL_AREA(#17580);
#17582=SURFACE_SIDE_STYLE('',(#17581));
#17583=SURFACE_STYLE_USAGE(.BOTH.,#17582);
#17584=PRESENTATION_STYLE_ASSIGNMENT((#17583));
ENDSEC;
END-ISO-10303-21;
